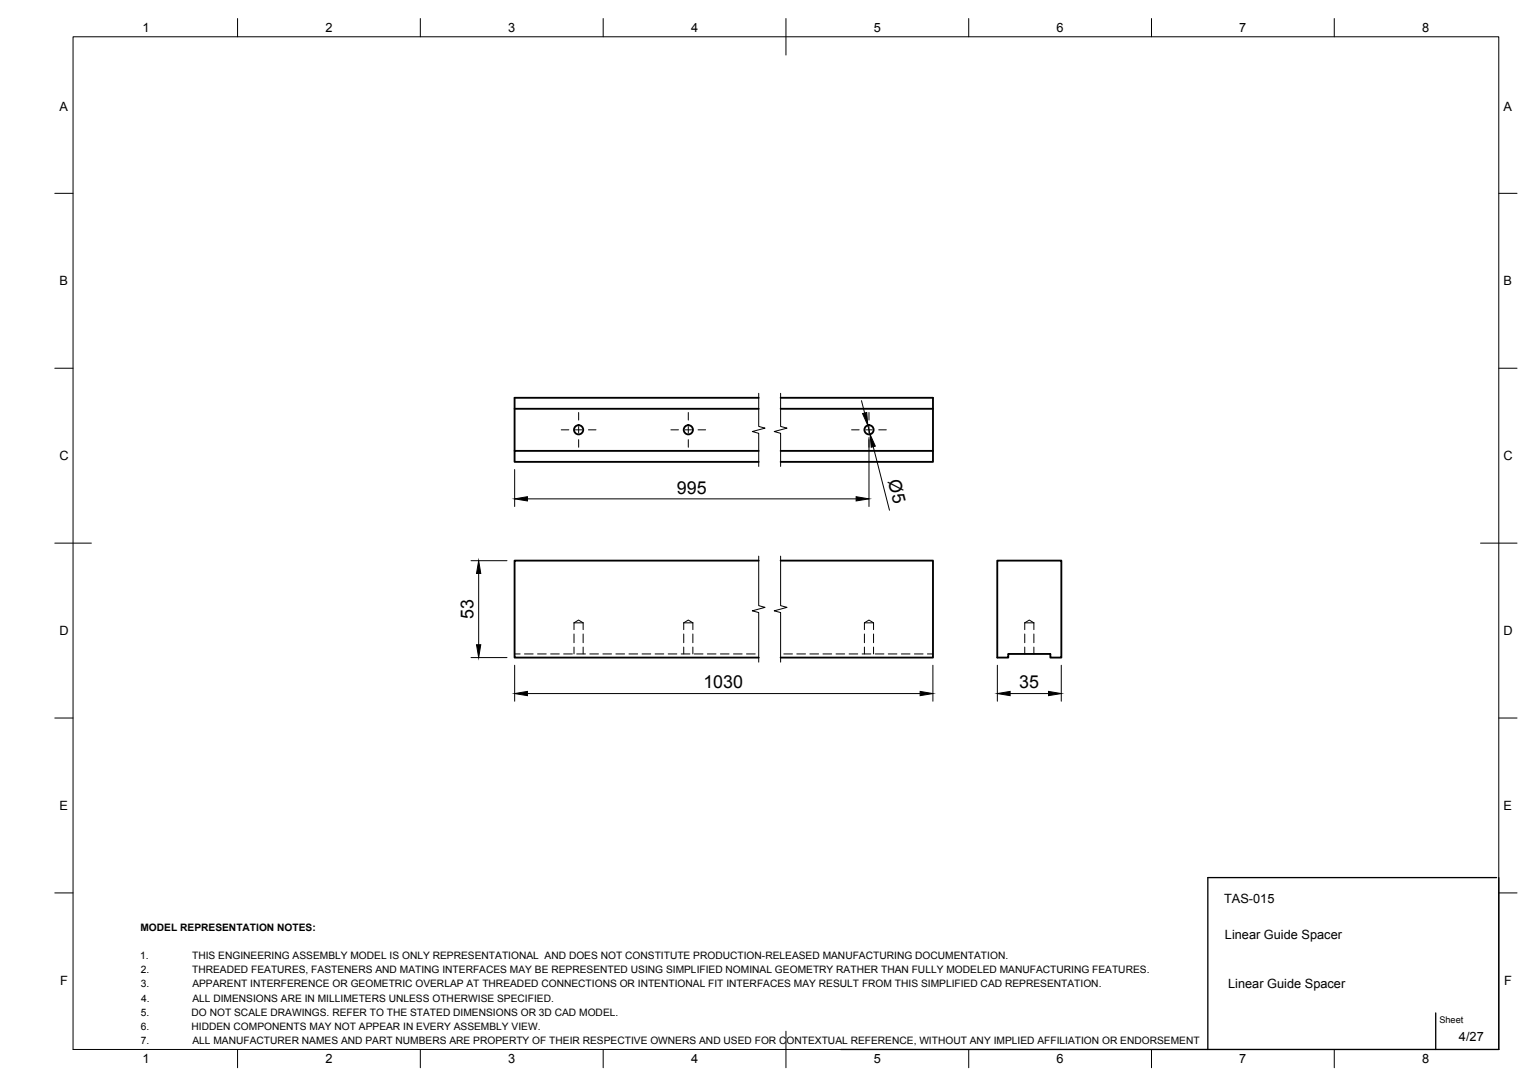
ISO-10303-21;
HEADER;
/* Generated by software containing ST-Developer
 * from STEP Tools, Inc. (www.steptools.com) 
 */

FILE_DESCRIPTION(
/* description */ ('STEP AP214'),
/* implementation_level */ '2;1');

FILE_NAME(
/* name */ 'Linear Guide Spacer.step',
/* time_stamp */ '2026-11-15T14:49:54-08:00',
/* author */ (''),
/* organization */ (''),
/* preprocessor_version */ 'ST-DEVELOPER v20.2',
/* originating_system */ 'Autodesk Translation Framework v15.17.0.0',
/* authorisation */ '');

FILE_SCHEMA (('AUTOMOTIVE_DESIGN { 1 0 10303 214 3 1 1 }'));
ENDSEC;

DATA;
#10=MECHANICAL_DESIGN_GEOMETRIC_PRESENTATION_REPRESENTATION('',(#1126),#66721);
#559=CONICAL_SURFACE('',#28483,2.5,1.02974425867665);
#560=CONICAL_SURFACE('',#28487,2.5,1.02974425867665);
#561=CONICAL_SURFACE('',#28491,2.5,1.02974425867665);
#562=CONICAL_SURFACE('',#28495,2.5,1.02974425867665);
#563=CONICAL_SURFACE('',#28499,2.5,1.02974425867665);
#564=CONICAL_SURFACE('',#28503,2.5,1.02974425867665);
#565=CONICAL_SURFACE('',#28507,2.5,1.02974425867665);
#566=CONICAL_SURFACE('',#28511,2.5,1.02974425867665);
#567=CONICAL_SURFACE('',#28515,2.5,1.02974425867665);
#568=CONICAL_SURFACE('',#28519,2.5,1.02974425867665);
#569=CONICAL_SURFACE('',#28523,2.5,1.02974425867665);
#570=CONICAL_SURFACE('',#28527,2.5,1.02974425867665);
#571=CONICAL_SURFACE('',#28531,2.5,1.02974425867665);
#572=CONICAL_SURFACE('',#28535,2.5,1.02974425867665);
#573=CONICAL_SURFACE('',#28539,2.5,1.02974425867665);
#574=CONICAL_SURFACE('',#28543,2.5,1.02974425867665);
#575=CONICAL_SURFACE('',#28547,2.5,1.02974425867665);
#1062=SHAPE_REPRESENTATION_RELATIONSHIP('SRR','None',#66925,#1093);
#1093=ADVANCED_BREP_SHAPE_REPRESENTATION('',(#1161),#66716);
#1126=STYLED_ITEM('',(#67095),#1161);
#1161=MANIFOLD_SOLID_BREP('Body1',#25692);
#1452=FACE_BOUND('',#5357,.T.);
#1453=FACE_BOUND('',#5358,.T.);
#1454=FACE_BOUND('',#5359,.T.);
#1455=FACE_BOUND('',#5360,.T.);
#1456=FACE_BOUND('',#5361,.T.);
#1457=FACE_BOUND('',#5362,.T.);
#1458=FACE_BOUND('',#5363,.T.);
#1459=FACE_BOUND('',#5364,.T.);
#1460=FACE_BOUND('',#5365,.T.);
#1461=FACE_BOUND('',#5366,.T.);
#1462=FACE_BOUND('',#5367,.T.);
#1463=FACE_BOUND('',#5368,.T.);
#1464=FACE_BOUND('',#5369,.T.);
#1465=FACE_BOUND('',#5370,.T.);
#1466=FACE_BOUND('',#5371,.T.);
#1467=FACE_BOUND('',#5372,.T.);
#1468=FACE_BOUND('',#5373,.T.);
#2209=PLANE('',#28548);
#2210=PLANE('',#28549);
#2211=PLANE('',#28552);
#2212=PLANE('',#28553);
#2213=PLANE('',#28556);
#2214=PLANE('',#28557);
#2215=PLANE('',#28558);
#2216=PLANE('',#28559);
#2217=PLANE('',#28560);
#2218=PLANE('',#28561);
#3588=FACE_OUTER_BOUND('',#5314,.T.);
#3589=FACE_OUTER_BOUND('',#5315,.T.);
#3590=FACE_OUTER_BOUND('',#5316,.T.);
#3591=FACE_OUTER_BOUND('',#5317,.T.);
#3592=FACE_OUTER_BOUND('',#5318,.T.);
#3593=FACE_OUTER_BOUND('',#5319,.T.);
#3594=FACE_OUTER_BOUND('',#5320,.T.);
#3595=FACE_OUTER_BOUND('',#5321,.T.);
#3596=FACE_OUTER_BOUND('',#5322,.T.);
#3597=FACE_OUTER_BOUND('',#5323,.T.);
#3598=FACE_OUTER_BOUND('',#5324,.T.);
#3599=FACE_OUTER_BOUND('',#5325,.T.);
#3600=FACE_OUTER_BOUND('',#5326,.T.);
#3601=FACE_OUTER_BOUND('',#5327,.T.);
#3602=FACE_OUTER_BOUND('',#5328,.T.);
#3603=FACE_OUTER_BOUND('',#5329,.T.);
#3604=FACE_OUTER_BOUND('',#5330,.T.);
#3605=FACE_OUTER_BOUND('',#5331,.T.);
#3606=FACE_OUTER_BOUND('',#5332,.T.);
#3607=FACE_OUTER_BOUND('',#5333,.T.);
#3608=FACE_OUTER_BOUND('',#5334,.T.);
#3609=FACE_OUTER_BOUND('',#5335,.T.);
#3610=FACE_OUTER_BOUND('',#5336,.T.);
#3611=FACE_OUTER_BOUND('',#5337,.T.);
#3612=FACE_OUTER_BOUND('',#5338,.T.);
#3613=FACE_OUTER_BOUND('',#5339,.T.);
#3614=FACE_OUTER_BOUND('',#5340,.T.);
#3615=FACE_OUTER_BOUND('',#5341,.T.);
#3616=FACE_OUTER_BOUND('',#5342,.T.);
#3617=FACE_OUTER_BOUND('',#5343,.T.);
#3618=FACE_OUTER_BOUND('',#5344,.T.);
#3619=FACE_OUTER_BOUND('',#5345,.T.);
#3620=FACE_OUTER_BOUND('',#5346,.T.);
#3621=FACE_OUTER_BOUND('',#5347,.T.);
#3622=FACE_OUTER_BOUND('',#5348,.T.);
#3623=FACE_OUTER_BOUND('',#5349,.T.);
#3624=FACE_OUTER_BOUND('',#5350,.T.);
#3625=FACE_OUTER_BOUND('',#5351,.T.);
#3626=FACE_OUTER_BOUND('',#5352,.T.);
#3627=FACE_OUTER_BOUND('',#5353,.T.);
#3628=FACE_OUTER_BOUND('',#5354,.T.);
#3629=FACE_OUTER_BOUND('',#5355,.T.);
#3630=FACE_OUTER_BOUND('',#5356,.T.);
#3631=FACE_OUTER_BOUND('',#5374,.T.);
#3632=FACE_OUTER_BOUND('',#5375,.T.);
#3633=FACE_OUTER_BOUND('',#5376,.T.);
#5314=EDGE_LOOP('',(#23270,#23271,#23272,#23273));
#5315=EDGE_LOOP('',(#23274,#23275,#23276));
#5316=EDGE_LOOP('',(#23277,#23278,#23279,#23280));
#5317=EDGE_LOOP('',(#23281,#23282,#23283));
#5318=EDGE_LOOP('',(#23284,#23285,#23286,#23287));
#5319=EDGE_LOOP('',(#23288,#23289,#23290));
#5320=EDGE_LOOP('',(#23291,#23292,#23293,#23294));
#5321=EDGE_LOOP('',(#23295,#23296,#23297));
#5322=EDGE_LOOP('',(#23298,#23299,#23300,#23301));
#5323=EDGE_LOOP('',(#23302,#23303,#23304));
#5324=EDGE_LOOP('',(#23305,#23306,#23307,#23308));
#5325=EDGE_LOOP('',(#23309,#23310,#23311));
#5326=EDGE_LOOP('',(#23312,#23313,#23314,#23315));
#5327=EDGE_LOOP('',(#23316,#23317,#23318));
#5328=EDGE_LOOP('',(#23319,#23320,#23321,#23322));
#5329=EDGE_LOOP('',(#23323,#23324,#23325));
#5330=EDGE_LOOP('',(#23326,#23327,#23328,#23329));
#5331=EDGE_LOOP('',(#23330,#23331,#23332));
#5332=EDGE_LOOP('',(#23333,#23334,#23335,#23336));
#5333=EDGE_LOOP('',(#23337,#23338,#23339));
#5334=EDGE_LOOP('',(#23340,#23341,#23342,#23343));
#5335=EDGE_LOOP('',(#23344,#23345,#23346));
#5336=EDGE_LOOP('',(#23347,#23348,#23349,#23350));
#5337=EDGE_LOOP('',(#23351,#23352,#23353));
#5338=EDGE_LOOP('',(#23354,#23355,#23356,#23357));
#5339=EDGE_LOOP('',(#23358,#23359,#23360));
#5340=EDGE_LOOP('',(#23361,#23362,#23363,#23364));
#5341=EDGE_LOOP('',(#23365,#23366,#23367));
#5342=EDGE_LOOP('',(#23368,#23369,#23370,#23371));
#5343=EDGE_LOOP('',(#23372,#23373,#23374));
#5344=EDGE_LOOP('',(#23375,#23376,#23377,#23378));
#5345=EDGE_LOOP('',(#23379,#23380,#23381));
#5346=EDGE_LOOP('',(#23382,#23383,#23384,#23385));
#5347=EDGE_LOOP('',(#23386,#23387,#23388));
#5348=EDGE_LOOP('',(#23389,#23390,#23391,#23392));
#5349=EDGE_LOOP('',(#23393,#23394,#23395,#23396,#23397,#23398,#23399,#23400,
#23401,#23402));
#5350=EDGE_LOOP('',(#23403,#23404,#23405,#23406));
#5351=EDGE_LOOP('',(#23407,#23408,#23409,#23410,#23411,#23412,#23413,#23414,
#23415,#23416));
#5352=EDGE_LOOP('',(#23417,#23418,#23419,#23420));
#5353=EDGE_LOOP('',(#23421,#23422,#23423,#23424));
#5354=EDGE_LOOP('',(#23425,#23426,#23427,#23428));
#5355=EDGE_LOOP('',(#23429,#23430,#23431,#23432));
#5356=EDGE_LOOP('',(#23433,#23434,#23435,#23436));
#5357=EDGE_LOOP('',(#23437));
#5358=EDGE_LOOP('',(#23438));
#5359=EDGE_LOOP('',(#23439));
#5360=EDGE_LOOP('',(#23440));
#5361=EDGE_LOOP('',(#23441));
#5362=EDGE_LOOP('',(#23442));
#5363=EDGE_LOOP('',(#23443));
#5364=EDGE_LOOP('',(#23444));
#5365=EDGE_LOOP('',(#23445));
#5366=EDGE_LOOP('',(#23446));
#5367=EDGE_LOOP('',(#23447));
#5368=EDGE_LOOP('',(#23448));
#5369=EDGE_LOOP('',(#23449));
#5370=EDGE_LOOP('',(#23450));
#5371=EDGE_LOOP('',(#23451));
#5372=EDGE_LOOP('',(#23452));
#5373=EDGE_LOOP('',(#23453));
#5374=EDGE_LOOP('',(#23454,#23455,#23456,#23457));
#5375=EDGE_LOOP('',(#23458,#23459,#23460,#23461));
#5376=EDGE_LOOP('',(#23462,#23463,#23464,#23465));
#7301=LINE('',#66016,#9290);
#7302=LINE('',#66020,#9291);
#7303=LINE('',#66025,#9292);
#7304=LINE('',#66029,#9293);
#7305=LINE('',#66034,#9294);
#7306=LINE('',#66038,#9295);
#7307=LINE('',#66043,#9296);
#7308=LINE('',#66047,#9297);
#7309=LINE('',#66052,#9298);
#7310=LINE('',#66056,#9299);
#7311=LINE('',#66061,#9300);
#7312=LINE('',#66065,#9301);
#7313=LINE('',#66070,#9302);
#7314=LINE('',#66074,#9303);
#7315=LINE('',#66079,#9304);
#7316=LINE('',#66083,#9305);
#7317=LINE('',#66088,#9306);
#7318=LINE('',#66092,#9307);
#7319=LINE('',#66097,#9308);
#7320=LINE('',#66101,#9309);
#7321=LINE('',#66106,#9310);
#7322=LINE('',#66110,#9311);
#7323=LINE('',#66115,#9312);
#7324=LINE('',#66119,#9313);
#7325=LINE('',#66124,#9314);
#7326=LINE('',#66128,#9315);
#7327=LINE('',#66133,#9316);
#7328=LINE('',#66137,#9317);
#7329=LINE('',#66142,#9318);
#7330=LINE('',#66146,#9319);
#7331=LINE('',#66151,#9320);
#7332=LINE('',#66155,#9321);
#7333=LINE('',#66160,#9322);
#7334=LINE('',#66164,#9323);
#7335=LINE('',#66168,#9324);
#7336=LINE('',#66170,#9325);
#7337=LINE('',#66172,#9326);
#7338=LINE('',#66173,#9327);
#7339=LINE('',#66176,#9328);
#7340=LINE('',#66180,#9329);
#7341=LINE('',#66184,#9330);
#7342=LINE('',#66186,#9331);
#7343=LINE('',#66188,#9332);
#7344=LINE('',#66190,#9333);
#7345=LINE('',#66191,#9334);
#7346=LINE('',#66194,#9335);
#7347=LINE('',#66196,#9336);
#7348=LINE('',#66197,#9337);
#7349=LINE('',#66201,#9338);
#7350=LINE('',#66205,#9339);
#7351=LINE('',#66208,#9340);
#7352=LINE('',#66209,#9341);
#7353=LINE('',#66211,#9342);
#7354=LINE('',#66212,#9343);
#7355=LINE('',#66214,#9344);
#7356=LINE('',#66215,#9345);
#7357=LINE('',#66219,#9346);
#7358=LINE('',#66221,#9347);
#7359=LINE('',#66222,#9348);
#7360=LINE('',#66224,#9349);
#9290=VECTOR('',#35456,2.5);
#9291=VECTOR('',#35461,2.5);
#9292=VECTOR('',#35466,2.5);
#9293=VECTOR('',#35471,2.5);
#9294=VECTOR('',#35476,2.5);
#9295=VECTOR('',#35481,2.5);
#9296=VECTOR('',#35486,2.5);
#9297=VECTOR('',#35491,2.5);
#9298=VECTOR('',#35496,2.5);
#9299=VECTOR('',#35501,2.5);
#9300=VECTOR('',#35506,2.5);
#9301=VECTOR('',#35511,2.5);
#9302=VECTOR('',#35516,2.5);
#9303=VECTOR('',#35521,2.5);
#9304=VECTOR('',#35526,2.5);
#9305=VECTOR('',#35531,2.5);
#9306=VECTOR('',#35536,2.5);
#9307=VECTOR('',#35541,2.5);
#9308=VECTOR('',#35546,2.5);
#9309=VECTOR('',#35551,2.5);
#9310=VECTOR('',#35556,2.5);
#9311=VECTOR('',#35561,2.5);
#9312=VECTOR('',#35566,2.5);
#9313=VECTOR('',#35571,2.5);
#9314=VECTOR('',#35576,2.5);
#9315=VECTOR('',#35581,2.5);
#9316=VECTOR('',#35586,2.5);
#9317=VECTOR('',#35591,2.5);
#9318=VECTOR('',#35596,2.5);
#9319=VECTOR('',#35601,2.5);
#9320=VECTOR('',#35606,2.5);
#9321=VECTOR('',#35611,2.5);
#9322=VECTOR('',#35616,2.5);
#9323=VECTOR('',#35621,2.5);
#9324=VECTOR('',#35624,1000.);
#9325=VECTOR('',#35625,1000.);
#9326=VECTOR('',#35626,1000.);
#9327=VECTOR('',#35627,1000.);
#9328=VECTOR('',#35630,1000.);
#9329=VECTOR('',#35633,1000.);
#9330=VECTOR('',#35636,1000.);
#9331=VECTOR('',#35637,1000.);
#9332=VECTOR('',#35638,1000.);
#9333=VECTOR('',#35639,1000.);
#9334=VECTOR('',#35640,1000.);
#9335=VECTOR('',#35643,1000.);
#9336=VECTOR('',#35644,1000.);
#9337=VECTOR('',#35645,1000.);
#9338=VECTOR('',#35648,1000.);
#9339=VECTOR('',#35651,1000.);
#9340=VECTOR('',#35654,1000.);
#9341=VECTOR('',#35655,1000.);
#9342=VECTOR('',#35656,1000.);
#9343=VECTOR('',#35657,1000.);
#9344=VECTOR('',#35660,1000.);
#9345=VECTOR('',#35661,1000.);
#9346=VECTOR('',#35668,1000.);
#9347=VECTOR('',#35671,1000.);
#9348=VECTOR('',#35672,1000.);
#9349=VECTOR('',#35675,1000.);
#10543=CIRCLE('',#28481,2.5);
#10544=CIRCLE('',#28482,2.5);
#10545=CIRCLE('',#28485,2.5);
#10546=CIRCLE('',#28486,2.5);
#10547=CIRCLE('',#28489,2.5);
#10548=CIRCLE('',#28490,2.5);
#10549=CIRCLE('',#28493,2.5);
#10550=CIRCLE('',#28494,2.5);
#10551=CIRCLE('',#28497,2.5);
#10552=CIRCLE('',#28498,2.5);
#10553=CIRCLE('',#28501,2.5);
#10554=CIRCLE('',#28502,2.5);
#10555=CIRCLE('',#28505,2.5);
#10556=CIRCLE('',#28506,2.5);
#10557=CIRCLE('',#28509,2.5);
#10558=CIRCLE('',#28510,2.5);
#10559=CIRCLE('',#28513,2.5);
#10560=CIRCLE('',#28514,2.5);
#10561=CIRCLE('',#28517,2.5);
#10562=CIRCLE('',#28518,2.5);
#10563=CIRCLE('',#28521,2.5);
#10564=CIRCLE('',#28522,2.5);
#10565=CIRCLE('',#28525,2.5);
#10566=CIRCLE('',#28526,2.5);
#10567=CIRCLE('',#28529,2.5);
#10568=CIRCLE('',#28530,2.5);
#10569=CIRCLE('',#28533,2.5);
#10570=CIRCLE('',#28534,2.5);
#10571=CIRCLE('',#28537,2.5);
#10572=CIRCLE('',#28538,2.5);
#10573=CIRCLE('',#28541,2.5);
#10574=CIRCLE('',#28542,2.5);
#10575=CIRCLE('',#28545,2.5);
#10576=CIRCLE('',#28546,2.5);
#10577=CIRCLE('',#28550,0.200000000000001);
#10578=CIRCLE('',#28551,0.200000000000001);
#10579=CIRCLE('',#28554,0.200000000000001);
#10580=CIRCLE('',#28555,0.200000000000001);
#12809=VERTEX_POINT('',#66013);
#12810=VERTEX_POINT('',#66015);
#12811=VERTEX_POINT('',#66019);
#12812=VERTEX_POINT('',#66022);
#12813=VERTEX_POINT('',#66024);
#12814=VERTEX_POINT('',#66028);
#12815=VERTEX_POINT('',#66031);
#12816=VERTEX_POINT('',#66033);
#12817=VERTEX_POINT('',#66037);
#12818=VERTEX_POINT('',#66040);
#12819=VERTEX_POINT('',#66042);
#12820=VERTEX_POINT('',#66046);
#12821=VERTEX_POINT('',#66049);
#12822=VERTEX_POINT('',#66051);
#12823=VERTEX_POINT('',#66055);
#12824=VERTEX_POINT('',#66058);
#12825=VERTEX_POINT('',#66060);
#12826=VERTEX_POINT('',#66064);
#12827=VERTEX_POINT('',#66067);
#12828=VERTEX_POINT('',#66069);
#12829=VERTEX_POINT('',#66073);
#12830=VERTEX_POINT('',#66076);
#12831=VERTEX_POINT('',#66078);
#12832=VERTEX_POINT('',#66082);
#12833=VERTEX_POINT('',#66085);
#12834=VERTEX_POINT('',#66087);
#12835=VERTEX_POINT('',#66091);
#12836=VERTEX_POINT('',#66094);
#12837=VERTEX_POINT('',#66096);
#12838=VERTEX_POINT('',#66100);
#12839=VERTEX_POINT('',#66103);
#12840=VERTEX_POINT('',#66105);
#12841=VERTEX_POINT('',#66109);
#12842=VERTEX_POINT('',#66112);
#12843=VERTEX_POINT('',#66114);
#12844=VERTEX_POINT('',#66118);
#12845=VERTEX_POINT('',#66121);
#12846=VERTEX_POINT('',#66123);
#12847=VERTEX_POINT('',#66127);
#12848=VERTEX_POINT('',#66130);
#12849=VERTEX_POINT('',#66132);
#12850=VERTEX_POINT('',#66136);
#12851=VERTEX_POINT('',#66139);
#12852=VERTEX_POINT('',#66141);
#12853=VERTEX_POINT('',#66145);
#12854=VERTEX_POINT('',#66148);
#12855=VERTEX_POINT('',#66150);
#12856=VERTEX_POINT('',#66154);
#12857=VERTEX_POINT('',#66157);
#12858=VERTEX_POINT('',#66159);
#12859=VERTEX_POINT('',#66163);
#12860=VERTEX_POINT('',#66166);
#12861=VERTEX_POINT('',#66167);
#12862=VERTEX_POINT('',#66169);
#12863=VERTEX_POINT('',#66171);
#12864=VERTEX_POINT('',#66175);
#12865=VERTEX_POINT('',#66177);
#12866=VERTEX_POINT('',#66179);
#12867=VERTEX_POINT('',#66181);
#12868=VERTEX_POINT('',#66183);
#12869=VERTEX_POINT('',#66185);
#12870=VERTEX_POINT('',#66187);
#12871=VERTEX_POINT('',#66189);
#12872=VERTEX_POINT('',#66193);
#12873=VERTEX_POINT('',#66195);
#12874=VERTEX_POINT('',#66199);
#12875=VERTEX_POINT('',#66200);
#12876=VERTEX_POINT('',#66202);
#12877=VERTEX_POINT('',#66204);
#12878=VERTEX_POINT('',#66206);
#12879=VERTEX_POINT('',#66210);
#16328=EDGE_CURVE('',#12809,#12809,#10543,.T.);
#16329=EDGE_CURVE('',#12809,#12810,#7301,.T.);
#16330=EDGE_CURVE('',#12810,#12810,#10544,.T.);
#16331=EDGE_CURVE('',#12811,#12809,#7302,.T.);
#16332=EDGE_CURVE('',#12812,#12812,#10545,.T.);
#16333=EDGE_CURVE('',#12812,#12813,#7303,.T.);
#16334=EDGE_CURVE('',#12813,#12813,#10546,.T.);
#16335=EDGE_CURVE('',#12814,#12812,#7304,.T.);
#16336=EDGE_CURVE('',#12815,#12815,#10547,.T.);
#16337=EDGE_CURVE('',#12815,#12816,#7305,.T.);
#16338=EDGE_CURVE('',#12816,#12816,#10548,.T.);
#16339=EDGE_CURVE('',#12817,#12815,#7306,.T.);
#16340=EDGE_CURVE('',#12818,#12818,#10549,.T.);
#16341=EDGE_CURVE('',#12818,#12819,#7307,.T.);
#16342=EDGE_CURVE('',#12819,#12819,#10550,.T.);
#16343=EDGE_CURVE('',#12820,#12818,#7308,.T.);
#16344=EDGE_CURVE('',#12821,#12821,#10551,.T.);
#16345=EDGE_CURVE('',#12821,#12822,#7309,.T.);
#16346=EDGE_CURVE('',#12822,#12822,#10552,.T.);
#16347=EDGE_CURVE('',#12823,#12821,#7310,.T.);
#16348=EDGE_CURVE('',#12824,#12824,#10553,.T.);
#16349=EDGE_CURVE('',#12824,#12825,#7311,.T.);
#16350=EDGE_CURVE('',#12825,#12825,#10554,.T.);
#16351=EDGE_CURVE('',#12826,#12824,#7312,.T.);
#16352=EDGE_CURVE('',#12827,#12827,#10555,.T.);
#16353=EDGE_CURVE('',#12827,#12828,#7313,.T.);
#16354=EDGE_CURVE('',#12828,#12828,#10556,.T.);
#16355=EDGE_CURVE('',#12829,#12827,#7314,.T.);
#16356=EDGE_CURVE('',#12830,#12830,#10557,.T.);
#16357=EDGE_CURVE('',#12830,#12831,#7315,.T.);
#16358=EDGE_CURVE('',#12831,#12831,#10558,.T.);
#16359=EDGE_CURVE('',#12832,#12830,#7316,.T.);
#16360=EDGE_CURVE('',#12833,#12833,#10559,.T.);
#16361=EDGE_CURVE('',#12833,#12834,#7317,.T.);
#16362=EDGE_CURVE('',#12834,#12834,#10560,.T.);
#16363=EDGE_CURVE('',#12835,#12833,#7318,.T.);
#16364=EDGE_CURVE('',#12836,#12836,#10561,.T.);
#16365=EDGE_CURVE('',#12836,#12837,#7319,.T.);
#16366=EDGE_CURVE('',#12837,#12837,#10562,.T.);
#16367=EDGE_CURVE('',#12838,#12836,#7320,.T.);
#16368=EDGE_CURVE('',#12839,#12839,#10563,.T.);
#16369=EDGE_CURVE('',#12839,#12840,#7321,.T.);
#16370=EDGE_CURVE('',#12840,#12840,#10564,.T.);
#16371=EDGE_CURVE('',#12841,#12839,#7322,.T.);
#16372=EDGE_CURVE('',#12842,#12842,#10565,.T.);
#16373=EDGE_CURVE('',#12842,#12843,#7323,.T.);
#16374=EDGE_CURVE('',#12843,#12843,#10566,.T.);
#16375=EDGE_CURVE('',#12844,#12842,#7324,.T.);
#16376=EDGE_CURVE('',#12845,#12845,#10567,.T.);
#16377=EDGE_CURVE('',#12845,#12846,#7325,.T.);
#16378=EDGE_CURVE('',#12846,#12846,#10568,.T.);
#16379=EDGE_CURVE('',#12847,#12845,#7326,.T.);
#16380=EDGE_CURVE('',#12848,#12848,#10569,.T.);
#16381=EDGE_CURVE('',#12848,#12849,#7327,.T.);
#16382=EDGE_CURVE('',#12849,#12849,#10570,.T.);
#16383=EDGE_CURVE('',#12850,#12848,#7328,.T.);
#16384=EDGE_CURVE('',#12851,#12851,#10571,.T.);
#16385=EDGE_CURVE('',#12851,#12852,#7329,.T.);
#16386=EDGE_CURVE('',#12852,#12852,#10572,.T.);
#16387=EDGE_CURVE('',#12853,#12851,#7330,.T.);
#16388=EDGE_CURVE('',#12854,#12854,#10573,.T.);
#16389=EDGE_CURVE('',#12854,#12855,#7331,.T.);
#16390=EDGE_CURVE('',#12855,#12855,#10574,.T.);
#16391=EDGE_CURVE('',#12856,#12854,#7332,.T.);
#16392=EDGE_CURVE('',#12857,#12857,#10575,.T.);
#16393=EDGE_CURVE('',#12857,#12858,#7333,.T.);
#16394=EDGE_CURVE('',#12858,#12858,#10576,.T.);
#16395=EDGE_CURVE('',#12859,#12857,#7334,.T.);
#16396=EDGE_CURVE('',#12860,#12861,#7335,.T.);
#16397=EDGE_CURVE('',#12861,#12862,#7336,.T.);
#16398=EDGE_CURVE('',#12863,#12862,#7337,.T.);
#16399=EDGE_CURVE('',#12860,#12863,#7338,.T.);
#16400=EDGE_CURVE('',#12864,#12862,#7339,.T.);
#16401=EDGE_CURVE('',#12864,#12865,#10577,.T.);
#16402=EDGE_CURVE('',#12866,#12865,#7340,.T.);
#16403=EDGE_CURVE('',#12866,#12867,#10578,.T.);
#16404=EDGE_CURVE('',#12868,#12867,#7341,.T.);
#16405=EDGE_CURVE('',#12868,#12869,#7342,.T.);
#16406=EDGE_CURVE('',#12869,#12870,#7343,.T.);
#16407=EDGE_CURVE('',#12871,#12870,#7344,.T.);
#16408=EDGE_CURVE('',#12863,#12871,#7345,.T.);
#16409=EDGE_CURVE('',#12870,#12872,#7346,.T.);
#16410=EDGE_CURVE('',#12873,#12872,#7347,.T.);
#16411=EDGE_CURVE('',#12871,#12873,#7348,.T.);
#16412=EDGE_CURVE('',#12874,#12875,#7349,.T.);
#16413=EDGE_CURVE('',#12875,#12876,#10579,.T.);
#16414=EDGE_CURVE('',#12876,#12877,#7350,.T.);
#16415=EDGE_CURVE('',#12877,#12878,#10580,.T.);
#16416=EDGE_CURVE('',#12878,#12861,#7351,.T.);
#16417=EDGE_CURVE('',#12873,#12860,#7352,.T.);
#16418=EDGE_CURVE('',#12872,#12879,#7353,.T.);
#16419=EDGE_CURVE('',#12874,#12879,#7354,.T.);
#16420=EDGE_CURVE('',#12874,#12868,#7355,.T.);
#16421=EDGE_CURVE('',#12879,#12869,#7356,.T.);
#16422=EDGE_CURVE('',#12878,#12864,#7357,.T.);
#16423=EDGE_CURVE('',#12876,#12866,#7358,.T.);
#16424=EDGE_CURVE('',#12865,#12877,#7359,.T.);
#16425=EDGE_CURVE('',#12867,#12875,#7360,.T.);
#23270=ORIENTED_EDGE('',*,*,#16328,.F.);
#23271=ORIENTED_EDGE('',*,*,#16329,.T.);
#23272=ORIENTED_EDGE('',*,*,#16330,.T.);
#23273=ORIENTED_EDGE('',*,*,#16329,.F.);
#23274=ORIENTED_EDGE('',*,*,#16331,.T.);
#23275=ORIENTED_EDGE('',*,*,#16328,.T.);
#23276=ORIENTED_EDGE('',*,*,#16331,.F.);
#23277=ORIENTED_EDGE('',*,*,#16332,.F.);
#23278=ORIENTED_EDGE('',*,*,#16333,.T.);
#23279=ORIENTED_EDGE('',*,*,#16334,.T.);
#23280=ORIENTED_EDGE('',*,*,#16333,.F.);
#23281=ORIENTED_EDGE('',*,*,#16335,.T.);
#23282=ORIENTED_EDGE('',*,*,#16332,.T.);
#23283=ORIENTED_EDGE('',*,*,#16335,.F.);
#23284=ORIENTED_EDGE('',*,*,#16336,.F.);
#23285=ORIENTED_EDGE('',*,*,#16337,.T.);
#23286=ORIENTED_EDGE('',*,*,#16338,.T.);
#23287=ORIENTED_EDGE('',*,*,#16337,.F.);
#23288=ORIENTED_EDGE('',*,*,#16339,.T.);
#23289=ORIENTED_EDGE('',*,*,#16336,.T.);
#23290=ORIENTED_EDGE('',*,*,#16339,.F.);
#23291=ORIENTED_EDGE('',*,*,#16340,.F.);
#23292=ORIENTED_EDGE('',*,*,#16341,.T.);
#23293=ORIENTED_EDGE('',*,*,#16342,.T.);
#23294=ORIENTED_EDGE('',*,*,#16341,.F.);
#23295=ORIENTED_EDGE('',*,*,#16343,.T.);
#23296=ORIENTED_EDGE('',*,*,#16340,.T.);
#23297=ORIENTED_EDGE('',*,*,#16343,.F.);
#23298=ORIENTED_EDGE('',*,*,#16344,.F.);
#23299=ORIENTED_EDGE('',*,*,#16345,.T.);
#23300=ORIENTED_EDGE('',*,*,#16346,.T.);
#23301=ORIENTED_EDGE('',*,*,#16345,.F.);
#23302=ORIENTED_EDGE('',*,*,#16347,.T.);
#23303=ORIENTED_EDGE('',*,*,#16344,.T.);
#23304=ORIENTED_EDGE('',*,*,#16347,.F.);
#23305=ORIENTED_EDGE('',*,*,#16348,.F.);
#23306=ORIENTED_EDGE('',*,*,#16349,.T.);
#23307=ORIENTED_EDGE('',*,*,#16350,.T.);
#23308=ORIENTED_EDGE('',*,*,#16349,.F.);
#23309=ORIENTED_EDGE('',*,*,#16351,.T.);
#23310=ORIENTED_EDGE('',*,*,#16348,.T.);
#23311=ORIENTED_EDGE('',*,*,#16351,.F.);
#23312=ORIENTED_EDGE('',*,*,#16352,.F.);
#23313=ORIENTED_EDGE('',*,*,#16353,.T.);
#23314=ORIENTED_EDGE('',*,*,#16354,.T.);
#23315=ORIENTED_EDGE('',*,*,#16353,.F.);
#23316=ORIENTED_EDGE('',*,*,#16355,.T.);
#23317=ORIENTED_EDGE('',*,*,#16352,.T.);
#23318=ORIENTED_EDGE('',*,*,#16355,.F.);
#23319=ORIENTED_EDGE('',*,*,#16356,.F.);
#23320=ORIENTED_EDGE('',*,*,#16357,.T.);
#23321=ORIENTED_EDGE('',*,*,#16358,.T.);
#23322=ORIENTED_EDGE('',*,*,#16357,.F.);
#23323=ORIENTED_EDGE('',*,*,#16359,.T.);
#23324=ORIENTED_EDGE('',*,*,#16356,.T.);
#23325=ORIENTED_EDGE('',*,*,#16359,.F.);
#23326=ORIENTED_EDGE('',*,*,#16360,.F.);
#23327=ORIENTED_EDGE('',*,*,#16361,.T.);
#23328=ORIENTED_EDGE('',*,*,#16362,.T.);
#23329=ORIENTED_EDGE('',*,*,#16361,.F.);
#23330=ORIENTED_EDGE('',*,*,#16363,.T.);
#23331=ORIENTED_EDGE('',*,*,#16360,.T.);
#23332=ORIENTED_EDGE('',*,*,#16363,.F.);
#23333=ORIENTED_EDGE('',*,*,#16364,.F.);
#23334=ORIENTED_EDGE('',*,*,#16365,.T.);
#23335=ORIENTED_EDGE('',*,*,#16366,.T.);
#23336=ORIENTED_EDGE('',*,*,#16365,.F.);
#23337=ORIENTED_EDGE('',*,*,#16367,.T.);
#23338=ORIENTED_EDGE('',*,*,#16364,.T.);
#23339=ORIENTED_EDGE('',*,*,#16367,.F.);
#23340=ORIENTED_EDGE('',*,*,#16368,.F.);
#23341=ORIENTED_EDGE('',*,*,#16369,.T.);
#23342=ORIENTED_EDGE('',*,*,#16370,.T.);
#23343=ORIENTED_EDGE('',*,*,#16369,.F.);
#23344=ORIENTED_EDGE('',*,*,#16371,.T.);
#23345=ORIENTED_EDGE('',*,*,#16368,.T.);
#23346=ORIENTED_EDGE('',*,*,#16371,.F.);
#23347=ORIENTED_EDGE('',*,*,#16372,.F.);
#23348=ORIENTED_EDGE('',*,*,#16373,.T.);
#23349=ORIENTED_EDGE('',*,*,#16374,.T.);
#23350=ORIENTED_EDGE('',*,*,#16373,.F.);
#23351=ORIENTED_EDGE('',*,*,#16375,.T.);
#23352=ORIENTED_EDGE('',*,*,#16372,.T.);
#23353=ORIENTED_EDGE('',*,*,#16375,.F.);
#23354=ORIENTED_EDGE('',*,*,#16376,.F.);
#23355=ORIENTED_EDGE('',*,*,#16377,.T.);
#23356=ORIENTED_EDGE('',*,*,#16378,.T.);
#23357=ORIENTED_EDGE('',*,*,#16377,.F.);
#23358=ORIENTED_EDGE('',*,*,#16379,.T.);
#23359=ORIENTED_EDGE('',*,*,#16376,.T.);
#23360=ORIENTED_EDGE('',*,*,#16379,.F.);
#23361=ORIENTED_EDGE('',*,*,#16380,.F.);
#23362=ORIENTED_EDGE('',*,*,#16381,.T.);
#23363=ORIENTED_EDGE('',*,*,#16382,.T.);
#23364=ORIENTED_EDGE('',*,*,#16381,.F.);
#23365=ORIENTED_EDGE('',*,*,#16383,.T.);
#23366=ORIENTED_EDGE('',*,*,#16380,.T.);
#23367=ORIENTED_EDGE('',*,*,#16383,.F.);
#23368=ORIENTED_EDGE('',*,*,#16384,.F.);
#23369=ORIENTED_EDGE('',*,*,#16385,.T.);
#23370=ORIENTED_EDGE('',*,*,#16386,.T.);
#23371=ORIENTED_EDGE('',*,*,#16385,.F.);
#23372=ORIENTED_EDGE('',*,*,#16387,.T.);
#23373=ORIENTED_EDGE('',*,*,#16384,.T.);
#23374=ORIENTED_EDGE('',*,*,#16387,.F.);
#23375=ORIENTED_EDGE('',*,*,#16388,.F.);
#23376=ORIENTED_EDGE('',*,*,#16389,.T.);
#23377=ORIENTED_EDGE('',*,*,#16390,.T.);
#23378=ORIENTED_EDGE('',*,*,#16389,.F.);
#23379=ORIENTED_EDGE('',*,*,#16391,.T.);
#23380=ORIENTED_EDGE('',*,*,#16388,.T.);
#23381=ORIENTED_EDGE('',*,*,#16391,.F.);
#23382=ORIENTED_EDGE('',*,*,#16392,.F.);
#23383=ORIENTED_EDGE('',*,*,#16393,.T.);
#23384=ORIENTED_EDGE('',*,*,#16394,.T.);
#23385=ORIENTED_EDGE('',*,*,#16393,.F.);
#23386=ORIENTED_EDGE('',*,*,#16395,.T.);
#23387=ORIENTED_EDGE('',*,*,#16392,.T.);
#23388=ORIENTED_EDGE('',*,*,#16395,.F.);
#23389=ORIENTED_EDGE('',*,*,#16396,.T.);
#23390=ORIENTED_EDGE('',*,*,#16397,.T.);
#23391=ORIENTED_EDGE('',*,*,#16398,.F.);
#23392=ORIENTED_EDGE('',*,*,#16399,.F.);
#23393=ORIENTED_EDGE('',*,*,#16398,.T.);
#23394=ORIENTED_EDGE('',*,*,#16400,.F.);
#23395=ORIENTED_EDGE('',*,*,#16401,.T.);
#23396=ORIENTED_EDGE('',*,*,#16402,.F.);
#23397=ORIENTED_EDGE('',*,*,#16403,.T.);
#23398=ORIENTED_EDGE('',*,*,#16404,.F.);
#23399=ORIENTED_EDGE('',*,*,#16405,.T.);
#23400=ORIENTED_EDGE('',*,*,#16406,.T.);
#23401=ORIENTED_EDGE('',*,*,#16407,.F.);
#23402=ORIENTED_EDGE('',*,*,#16408,.F.);
#23403=ORIENTED_EDGE('',*,*,#16409,.T.);
#23404=ORIENTED_EDGE('',*,*,#16410,.F.);
#23405=ORIENTED_EDGE('',*,*,#16411,.F.);
#23406=ORIENTED_EDGE('',*,*,#16407,.T.);
#23407=ORIENTED_EDGE('',*,*,#16412,.T.);
#23408=ORIENTED_EDGE('',*,*,#16413,.T.);
#23409=ORIENTED_EDGE('',*,*,#16414,.T.);
#23410=ORIENTED_EDGE('',*,*,#16415,.T.);
#23411=ORIENTED_EDGE('',*,*,#16416,.T.);
#23412=ORIENTED_EDGE('',*,*,#16396,.F.);
#23413=ORIENTED_EDGE('',*,*,#16417,.F.);
#23414=ORIENTED_EDGE('',*,*,#16410,.T.);
#23415=ORIENTED_EDGE('',*,*,#16418,.T.);
#23416=ORIENTED_EDGE('',*,*,#16419,.F.);
#23417=ORIENTED_EDGE('',*,*,#16405,.F.);
#23418=ORIENTED_EDGE('',*,*,#16420,.F.);
#23419=ORIENTED_EDGE('',*,*,#16419,.T.);
#23420=ORIENTED_EDGE('',*,*,#16421,.T.);
#23421=ORIENTED_EDGE('',*,*,#16408,.T.);
#23422=ORIENTED_EDGE('',*,*,#16411,.T.);
#23423=ORIENTED_EDGE('',*,*,#16417,.T.);
#23424=ORIENTED_EDGE('',*,*,#16399,.T.);
#23425=ORIENTED_EDGE('',*,*,#16406,.F.);
#23426=ORIENTED_EDGE('',*,*,#16421,.F.);
#23427=ORIENTED_EDGE('',*,*,#16418,.F.);
#23428=ORIENTED_EDGE('',*,*,#16409,.F.);
#23429=ORIENTED_EDGE('',*,*,#16416,.F.);
#23430=ORIENTED_EDGE('',*,*,#16422,.T.);
#23431=ORIENTED_EDGE('',*,*,#16400,.T.);
#23432=ORIENTED_EDGE('',*,*,#16397,.F.);
#23433=ORIENTED_EDGE('',*,*,#16414,.F.);
#23434=ORIENTED_EDGE('',*,*,#16423,.T.);
#23435=ORIENTED_EDGE('',*,*,#16402,.T.);
#23436=ORIENTED_EDGE('',*,*,#16424,.T.);
#23437=ORIENTED_EDGE('',*,*,#16330,.F.);
#23438=ORIENTED_EDGE('',*,*,#16334,.F.);
#23439=ORIENTED_EDGE('',*,*,#16338,.F.);
#23440=ORIENTED_EDGE('',*,*,#16342,.F.);
#23441=ORIENTED_EDGE('',*,*,#16346,.F.);
#23442=ORIENTED_EDGE('',*,*,#16350,.F.);
#23443=ORIENTED_EDGE('',*,*,#16354,.F.);
#23444=ORIENTED_EDGE('',*,*,#16358,.F.);
#23445=ORIENTED_EDGE('',*,*,#16362,.F.);
#23446=ORIENTED_EDGE('',*,*,#16366,.F.);
#23447=ORIENTED_EDGE('',*,*,#16370,.F.);
#23448=ORIENTED_EDGE('',*,*,#16374,.F.);
#23449=ORIENTED_EDGE('',*,*,#16378,.F.);
#23450=ORIENTED_EDGE('',*,*,#16382,.F.);
#23451=ORIENTED_EDGE('',*,*,#16386,.F.);
#23452=ORIENTED_EDGE('',*,*,#16390,.F.);
#23453=ORIENTED_EDGE('',*,*,#16394,.F.);
#23454=ORIENTED_EDGE('',*,*,#16404,.T.);
#23455=ORIENTED_EDGE('',*,*,#16425,.T.);
#23456=ORIENTED_EDGE('',*,*,#16412,.F.);
#23457=ORIENTED_EDGE('',*,*,#16420,.T.);
#23458=ORIENTED_EDGE('',*,*,#16413,.F.);
#23459=ORIENTED_EDGE('',*,*,#16425,.F.);
#23460=ORIENTED_EDGE('',*,*,#16403,.F.);
#23461=ORIENTED_EDGE('',*,*,#16423,.F.);
#23462=ORIENTED_EDGE('',*,*,#16415,.F.);
#23463=ORIENTED_EDGE('',*,*,#16424,.F.);
#23464=ORIENTED_EDGE('',*,*,#16401,.F.);
#23465=ORIENTED_EDGE('',*,*,#16422,.F.);
#24182=CYLINDRICAL_SURFACE('',#28480,2.5);
#24183=CYLINDRICAL_SURFACE('',#28484,2.5);
#24184=CYLINDRICAL_SURFACE('',#28488,2.5);
#24185=CYLINDRICAL_SURFACE('',#28492,2.5);
#24186=CYLINDRICAL_SURFACE('',#28496,2.5);
#24187=CYLINDRICAL_SURFACE('',#28500,2.5);
#24188=CYLINDRICAL_SURFACE('',#28504,2.5);
#24189=CYLINDRICAL_SURFACE('',#28508,2.5);
#24190=CYLINDRICAL_SURFACE('',#28512,2.5);
#24191=CYLINDRICAL_SURFACE('',#28516,2.5);
#24192=CYLINDRICAL_SURFACE('',#28520,2.5);
#24193=CYLINDRICAL_SURFACE('',#28524,2.5);
#24194=CYLINDRICAL_SURFACE('',#28528,2.5);
#24195=CYLINDRICAL_SURFACE('',#28532,2.5);
#24196=CYLINDRICAL_SURFACE('',#28536,2.5);
#24197=CYLINDRICAL_SURFACE('',#28540,2.5);
#24198=CYLINDRICAL_SURFACE('',#28544,2.5);
#24199=CYLINDRICAL_SURFACE('',#28562,0.200000000000001);
#24200=CYLINDRICAL_SURFACE('',#28563,0.200000000000001);
#25541=ADVANCED_FACE('',(#3588),#24182,.F.);
#25542=ADVANCED_FACE('',(#3589),#559,.F.);
#25543=ADVANCED_FACE('',(#3590),#24183,.F.);
#25544=ADVANCED_FACE('',(#3591),#560,.F.);
#25545=ADVANCED_FACE('',(#3592),#24184,.F.);
#25546=ADVANCED_FACE('',(#3593),#561,.F.);
#25547=ADVANCED_FACE('',(#3594),#24185,.F.);
#25548=ADVANCED_FACE('',(#3595),#562,.F.);
#25549=ADVANCED_FACE('',(#3596),#24186,.F.);
#25550=ADVANCED_FACE('',(#3597),#563,.F.);
#25551=ADVANCED_FACE('',(#3598),#24187,.F.);
#25552=ADVANCED_FACE('',(#3599),#564,.F.);
#25553=ADVANCED_FACE('',(#3600),#24188,.F.);
#25554=ADVANCED_FACE('',(#3601),#565,.F.);
#25555=ADVANCED_FACE('',(#3602),#24189,.F.);
#25556=ADVANCED_FACE('',(#3603),#566,.F.);
#25557=ADVANCED_FACE('',(#3604),#24190,.F.);
#25558=ADVANCED_FACE('',(#3605),#567,.F.);
#25559=ADVANCED_FACE('',(#3606),#24191,.F.);
#25560=ADVANCED_FACE('',(#3607),#568,.F.);
#25561=ADVANCED_FACE('',(#3608),#24192,.F.);
#25562=ADVANCED_FACE('',(#3609),#569,.F.);
#25563=ADVANCED_FACE('',(#3610),#24193,.F.);
#25564=ADVANCED_FACE('',(#3611),#570,.F.);
#25565=ADVANCED_FACE('',(#3612),#24194,.F.);
#25566=ADVANCED_FACE('',(#3613),#571,.F.);
#25567=ADVANCED_FACE('',(#3614),#24195,.F.);
#25568=ADVANCED_FACE('',(#3615),#572,.F.);
#25569=ADVANCED_FACE('',(#3616),#24196,.F.);
#25570=ADVANCED_FACE('',(#3617),#573,.F.);
#25571=ADVANCED_FACE('',(#3618),#24197,.F.);
#25572=ADVANCED_FACE('',(#3619),#574,.F.);
#25573=ADVANCED_FACE('',(#3620),#24198,.F.);
#25574=ADVANCED_FACE('',(#3621),#575,.F.);
#25575=ADVANCED_FACE('',(#3622),#2209,.F.);
#25576=ADVANCED_FACE('',(#3623),#2210,.F.);
#25577=ADVANCED_FACE('',(#3624),#2211,.F.);
#25578=ADVANCED_FACE('',(#3625),#2212,.F.);
#25579=ADVANCED_FACE('',(#3626),#2213,.F.);
#25580=ADVANCED_FACE('',(#3627),#2214,.T.);
#25581=ADVANCED_FACE('',(#3628),#2215,.F.);
#25582=ADVANCED_FACE('',(#3629),#2216,.F.);
#25583=ADVANCED_FACE('',(#3630,#1452,#1453,#1454,#1455,#1456,#1457,#1458,
#1459,#1460,#1461,#1462,#1463,#1464,#1465,#1466,#1467,#1468),#2217,.F.);
#25584=ADVANCED_FACE('',(#3631),#2218,.F.);
#25585=ADVANCED_FACE('',(#3632),#24199,.F.);
#25586=ADVANCED_FACE('',(#3633),#24200,.F.);
#25692=CLOSED_SHELL('',(#25541,#25542,#25543,#25544,#25545,#25546,#25547,
#25548,#25549,#25550,#25551,#25552,#25553,#25554,#25555,#25556,#25557,#25558,
#25559,#25560,#25561,#25562,#25563,#25564,#25565,#25566,#25567,#25568,#25569,
#25570,#25571,#25572,#25573,#25574,#25575,#25576,#25577,#25578,#25579,#25580,
#25581,#25582,#25583,#25584,#25585,#25586));
#28479=AXIS2_PLACEMENT_3D('',#66011,#35450,#35451);
#28480=AXIS2_PLACEMENT_3D('',#66012,#35452,#35453);
#28481=AXIS2_PLACEMENT_3D('',#66014,#35454,#35455);
#28482=AXIS2_PLACEMENT_3D('',#66017,#35457,#35458);
#28483=AXIS2_PLACEMENT_3D('',#66018,#35459,#35460);
#28484=AXIS2_PLACEMENT_3D('',#66021,#35462,#35463);
#28485=AXIS2_PLACEMENT_3D('',#66023,#35464,#35465);
#28486=AXIS2_PLACEMENT_3D('',#66026,#35467,#35468);
#28487=AXIS2_PLACEMENT_3D('',#66027,#35469,#35470);
#28488=AXIS2_PLACEMENT_3D('',#66030,#35472,#35473);
#28489=AXIS2_PLACEMENT_3D('',#66032,#35474,#35475);
#28490=AXIS2_PLACEMENT_3D('',#66035,#35477,#35478);
#28491=AXIS2_PLACEMENT_3D('',#66036,#35479,#35480);
#28492=AXIS2_PLACEMENT_3D('',#66039,#35482,#35483);
#28493=AXIS2_PLACEMENT_3D('',#66041,#35484,#35485);
#28494=AXIS2_PLACEMENT_3D('',#66044,#35487,#35488);
#28495=AXIS2_PLACEMENT_3D('',#66045,#35489,#35490);
#28496=AXIS2_PLACEMENT_3D('',#66048,#35492,#35493);
#28497=AXIS2_PLACEMENT_3D('',#66050,#35494,#35495);
#28498=AXIS2_PLACEMENT_3D('',#66053,#35497,#35498);
#28499=AXIS2_PLACEMENT_3D('',#66054,#35499,#35500);
#28500=AXIS2_PLACEMENT_3D('',#66057,#35502,#35503);
#28501=AXIS2_PLACEMENT_3D('',#66059,#35504,#35505);
#28502=AXIS2_PLACEMENT_3D('',#66062,#35507,#35508);
#28503=AXIS2_PLACEMENT_3D('',#66063,#35509,#35510);
#28504=AXIS2_PLACEMENT_3D('',#66066,#35512,#35513);
#28505=AXIS2_PLACEMENT_3D('',#66068,#35514,#35515);
#28506=AXIS2_PLACEMENT_3D('',#66071,#35517,#35518);
#28507=AXIS2_PLACEMENT_3D('',#66072,#35519,#35520);
#28508=AXIS2_PLACEMENT_3D('',#66075,#35522,#35523);
#28509=AXIS2_PLACEMENT_3D('',#66077,#35524,#35525);
#28510=AXIS2_PLACEMENT_3D('',#66080,#35527,#35528);
#28511=AXIS2_PLACEMENT_3D('',#66081,#35529,#35530);
#28512=AXIS2_PLACEMENT_3D('',#66084,#35532,#35533);
#28513=AXIS2_PLACEMENT_3D('',#66086,#35534,#35535);
#28514=AXIS2_PLACEMENT_3D('',#66089,#35537,#35538);
#28515=AXIS2_PLACEMENT_3D('',#66090,#35539,#35540);
#28516=AXIS2_PLACEMENT_3D('',#66093,#35542,#35543);
#28517=AXIS2_PLACEMENT_3D('',#66095,#35544,#35545);
#28518=AXIS2_PLACEMENT_3D('',#66098,#35547,#35548);
#28519=AXIS2_PLACEMENT_3D('',#66099,#35549,#35550);
#28520=AXIS2_PLACEMENT_3D('',#66102,#35552,#35553);
#28521=AXIS2_PLACEMENT_3D('',#66104,#35554,#35555);
#28522=AXIS2_PLACEMENT_3D('',#66107,#35557,#35558);
#28523=AXIS2_PLACEMENT_3D('',#66108,#35559,#35560);
#28524=AXIS2_PLACEMENT_3D('',#66111,#35562,#35563);
#28525=AXIS2_PLACEMENT_3D('',#66113,#35564,#35565);
#28526=AXIS2_PLACEMENT_3D('',#66116,#35567,#35568);
#28527=AXIS2_PLACEMENT_3D('',#66117,#35569,#35570);
#28528=AXIS2_PLACEMENT_3D('',#66120,#35572,#35573);
#28529=AXIS2_PLACEMENT_3D('',#66122,#35574,#35575);
#28530=AXIS2_PLACEMENT_3D('',#66125,#35577,#35578);
#28531=AXIS2_PLACEMENT_3D('',#66126,#35579,#35580);
#28532=AXIS2_PLACEMENT_3D('',#66129,#35582,#35583);
#28533=AXIS2_PLACEMENT_3D('',#66131,#35584,#35585);
#28534=AXIS2_PLACEMENT_3D('',#66134,#35587,#35588);
#28535=AXIS2_PLACEMENT_3D('',#66135,#35589,#35590);
#28536=AXIS2_PLACEMENT_3D('',#66138,#35592,#35593);
#28537=AXIS2_PLACEMENT_3D('',#66140,#35594,#35595);
#28538=AXIS2_PLACEMENT_3D('',#66143,#35597,#35598);
#28539=AXIS2_PLACEMENT_3D('',#66144,#35599,#35600);
#28540=AXIS2_PLACEMENT_3D('',#66147,#35602,#35603);
#28541=AXIS2_PLACEMENT_3D('',#66149,#35604,#35605);
#28542=AXIS2_PLACEMENT_3D('',#66152,#35607,#35608);
#28543=AXIS2_PLACEMENT_3D('',#66153,#35609,#35610);
#28544=AXIS2_PLACEMENT_3D('',#66156,#35612,#35613);
#28545=AXIS2_PLACEMENT_3D('',#66158,#35614,#35615);
#28546=AXIS2_PLACEMENT_3D('',#66161,#35617,#35618);
#28547=AXIS2_PLACEMENT_3D('',#66162,#35619,#35620);
#28548=AXIS2_PLACEMENT_3D('',#66165,#35622,#35623);
#28549=AXIS2_PLACEMENT_3D('',#66174,#35628,#35629);
#28550=AXIS2_PLACEMENT_3D('',#66178,#35631,#35632);
#28551=AXIS2_PLACEMENT_3D('',#66182,#35634,#35635);
#28552=AXIS2_PLACEMENT_3D('',#66192,#35641,#35642);
#28553=AXIS2_PLACEMENT_3D('',#66198,#35646,#35647);
#28554=AXIS2_PLACEMENT_3D('',#66203,#35649,#35650);
#28555=AXIS2_PLACEMENT_3D('',#66207,#35652,#35653);
#28556=AXIS2_PLACEMENT_3D('',#66213,#35658,#35659);
#28557=AXIS2_PLACEMENT_3D('',#66216,#35662,#35663);
#28558=AXIS2_PLACEMENT_3D('',#66217,#35664,#35665);
#28559=AXIS2_PLACEMENT_3D('',#66218,#35666,#35667);
#28560=AXIS2_PLACEMENT_3D('',#66220,#35669,#35670);
#28561=AXIS2_PLACEMENT_3D('',#66223,#35673,#35674);
#28562=AXIS2_PLACEMENT_3D('',#66225,#35676,#35677);
#28563=AXIS2_PLACEMENT_3D('',#66226,#35678,#35679);
#35450=DIRECTION('axis',(0.,0.,1.));
#35451=DIRECTION('refdir',(1.,0.,0.));
#35452=DIRECTION('center_axis',(0.,-1.,0.));
#35453=DIRECTION('ref_axis',(0.,0.,-1.));
#35454=DIRECTION('center_axis',(0.,-1.,0.));
#35455=DIRECTION('ref_axis',(0.,0.,-1.));
#35456=DIRECTION('',(0.,-1.,0.));
#35457=DIRECTION('center_axis',(0.,-1.,0.));
#35458=DIRECTION('ref_axis',(0.,0.,-1.));
#35459=DIRECTION('center_axis',(0.,-1.,0.));
#35460=DIRECTION('ref_axis',(0.,0.,-1.));
#35461=DIRECTION('',(-1.04972719113862E-16,-0.515038074910054,0.857167300702112));
#35462=DIRECTION('center_axis',(0.,-1.,0.));
#35463=DIRECTION('ref_axis',(0.,0.,-1.));
#35464=DIRECTION('center_axis',(0.,-1.,0.));
#35465=DIRECTION('ref_axis',(0.,0.,-1.));
#35466=DIRECTION('',(0.,-1.,0.));
#35467=DIRECTION('center_axis',(0.,-1.,0.));
#35468=DIRECTION('ref_axis',(0.,0.,-1.));
#35469=DIRECTION('center_axis',(0.,-1.,0.));
#35470=DIRECTION('ref_axis',(0.,0.,-1.));
#35471=DIRECTION('',(-1.04972719113862E-16,-0.515038074910054,0.857167300702112));
#35472=DIRECTION('center_axis',(0.,-1.,0.));
#35473=DIRECTION('ref_axis',(0.,0.,-1.));
#35474=DIRECTION('center_axis',(0.,-1.,0.));
#35475=DIRECTION('ref_axis',(0.,0.,-1.));
#35476=DIRECTION('',(0.,-1.,0.));
#35477=DIRECTION('center_axis',(0.,-1.,0.));
#35478=DIRECTION('ref_axis',(0.,0.,-1.));
#35479=DIRECTION('center_axis',(0.,-1.,0.));
#35480=DIRECTION('ref_axis',(0.,0.,-1.));
#35481=DIRECTION('',(-1.04972719113862E-16,-0.515038074910054,0.857167300702112));
#35482=DIRECTION('center_axis',(0.,-1.,0.));
#35483=DIRECTION('ref_axis',(0.,0.,-1.));
#35484=DIRECTION('center_axis',(0.,-1.,0.));
#35485=DIRECTION('ref_axis',(0.,0.,-1.));
#35486=DIRECTION('',(0.,-1.,0.));
#35487=DIRECTION('center_axis',(0.,-1.,0.));
#35488=DIRECTION('ref_axis',(0.,0.,-1.));
#35489=DIRECTION('center_axis',(0.,-1.,0.));
#35490=DIRECTION('ref_axis',(0.,0.,-1.));
#35491=DIRECTION('',(-1.04972719113862E-16,-0.515038074910054,0.857167300702112));
#35492=DIRECTION('center_axis',(0.,-1.,0.));
#35493=DIRECTION('ref_axis',(0.,0.,-1.));
#35494=DIRECTION('center_axis',(0.,-1.,0.));
#35495=DIRECTION('ref_axis',(0.,0.,-1.));
#35496=DIRECTION('',(0.,-1.,0.));
#35497=DIRECTION('center_axis',(0.,-1.,0.));
#35498=DIRECTION('ref_axis',(0.,0.,-1.));
#35499=DIRECTION('center_axis',(0.,-1.,0.));
#35500=DIRECTION('ref_axis',(0.,0.,-1.));
#35501=DIRECTION('',(-1.04972719113862E-16,-0.515038074910054,0.857167300702112));
#35502=DIRECTION('center_axis',(0.,-1.,0.));
#35503=DIRECTION('ref_axis',(0.,0.,-1.));
#35504=DIRECTION('center_axis',(0.,-1.,0.));
#35505=DIRECTION('ref_axis',(0.,0.,-1.));
#35506=DIRECTION('',(0.,-1.,0.));
#35507=DIRECTION('center_axis',(0.,-1.,0.));
#35508=DIRECTION('ref_axis',(0.,0.,-1.));
#35509=DIRECTION('center_axis',(0.,-1.,0.));
#35510=DIRECTION('ref_axis',(0.,0.,-1.));
#35511=DIRECTION('',(-1.04972719113862E-16,-0.515038074910054,0.857167300702112));
#35512=DIRECTION('center_axis',(0.,-1.,0.));
#35513=DIRECTION('ref_axis',(0.,0.,-1.));
#35514=DIRECTION('center_axis',(0.,-1.,0.));
#35515=DIRECTION('ref_axis',(0.,0.,-1.));
#35516=DIRECTION('',(0.,-1.,0.));
#35517=DIRECTION('center_axis',(0.,-1.,0.));
#35518=DIRECTION('ref_axis',(0.,0.,-1.));
#35519=DIRECTION('center_axis',(0.,-1.,0.));
#35520=DIRECTION('ref_axis',(0.,0.,-1.));
#35521=DIRECTION('',(-1.04972719113862E-16,-0.515038074910054,0.857167300702112));
#35522=DIRECTION('center_axis',(0.,-1.,0.));
#35523=DIRECTION('ref_axis',(0.,0.,-1.));
#35524=DIRECTION('center_axis',(0.,-1.,0.));
#35525=DIRECTION('ref_axis',(0.,0.,-1.));
#35526=DIRECTION('',(0.,-1.,0.));
#35527=DIRECTION('center_axis',(0.,-1.,0.));
#35528=DIRECTION('ref_axis',(0.,0.,-1.));
#35529=DIRECTION('center_axis',(0.,-1.,0.));
#35530=DIRECTION('ref_axis',(0.,0.,-1.));
#35531=DIRECTION('',(-1.04972719113862E-16,-0.515038074910057,0.857167300702111));
#35532=DIRECTION('center_axis',(0.,-1.,0.));
#35533=DIRECTION('ref_axis',(0.,0.,-1.));
#35534=DIRECTION('center_axis',(0.,-1.,0.));
#35535=DIRECTION('ref_axis',(0.,0.,-1.));
#35536=DIRECTION('',(0.,-1.,0.));
#35537=DIRECTION('center_axis',(0.,-1.,0.));
#35538=DIRECTION('ref_axis',(0.,0.,-1.));
#35539=DIRECTION('center_axis',(0.,-1.,0.));
#35540=DIRECTION('ref_axis',(0.,0.,-1.));
#35541=DIRECTION('',(-1.04972719113862E-16,-0.515038074910054,0.857167300702112));
#35542=DIRECTION('center_axis',(0.,-1.,0.));
#35543=DIRECTION('ref_axis',(0.,0.,-1.));
#35544=DIRECTION('center_axis',(0.,-1.,0.));
#35545=DIRECTION('ref_axis',(0.,0.,-1.));
#35546=DIRECTION('',(0.,-1.,0.));
#35547=DIRECTION('center_axis',(0.,-1.,0.));
#35548=DIRECTION('ref_axis',(0.,0.,-1.));
#35549=DIRECTION('center_axis',(0.,-1.,0.));
#35550=DIRECTION('ref_axis',(0.,0.,-1.));
#35551=DIRECTION('',(-1.04972719113862E-16,-0.515038074910054,0.857167300702112));
#35552=DIRECTION('center_axis',(0.,-1.,0.));
#35553=DIRECTION('ref_axis',(0.,0.,-1.));
#35554=DIRECTION('center_axis',(0.,-1.,0.));
#35555=DIRECTION('ref_axis',(0.,0.,-1.));
#35556=DIRECTION('',(0.,-1.,0.));
#35557=DIRECTION('center_axis',(0.,-1.,0.));
#35558=DIRECTION('ref_axis',(0.,0.,-1.));
#35559=DIRECTION('center_axis',(0.,-1.,0.));
#35560=DIRECTION('ref_axis',(0.,0.,-1.));
#35561=DIRECTION('',(-1.04972719113862E-16,-0.515038074910054,0.857167300702112));
#35562=DIRECTION('center_axis',(0.,-1.,0.));
#35563=DIRECTION('ref_axis',(0.,0.,-1.));
#35564=DIRECTION('center_axis',(0.,-1.,0.));
#35565=DIRECTION('ref_axis',(0.,0.,-1.));
#35566=DIRECTION('',(0.,-1.,0.));
#35567=DIRECTION('center_axis',(0.,-1.,0.));
#35568=DIRECTION('ref_axis',(0.,0.,-1.));
#35569=DIRECTION('center_axis',(0.,-1.,0.));
#35570=DIRECTION('ref_axis',(0.,0.,-1.));
#35571=DIRECTION('',(-1.04972719113862E-16,-0.515038074910054,0.857167300702112));
#35572=DIRECTION('center_axis',(0.,-1.,0.));
#35573=DIRECTION('ref_axis',(0.,0.,-1.));
#35574=DIRECTION('center_axis',(0.,-1.,0.));
#35575=DIRECTION('ref_axis',(0.,0.,-1.));
#35576=DIRECTION('',(0.,-1.,0.));
#35577=DIRECTION('center_axis',(0.,-1.,0.));
#35578=DIRECTION('ref_axis',(0.,0.,-1.));
#35579=DIRECTION('center_axis',(0.,-1.,0.));
#35580=DIRECTION('ref_axis',(0.,0.,-1.));
#35581=DIRECTION('',(-1.04972719113862E-16,-0.515038074910054,0.857167300702112));
#35582=DIRECTION('center_axis',(0.,-1.,0.));
#35583=DIRECTION('ref_axis',(0.,0.,-1.));
#35584=DIRECTION('center_axis',(0.,-1.,0.));
#35585=DIRECTION('ref_axis',(0.,0.,-1.));
#35586=DIRECTION('',(0.,-1.,0.));
#35587=DIRECTION('center_axis',(0.,-1.,0.));
#35588=DIRECTION('ref_axis',(0.,0.,-1.));
#35589=DIRECTION('center_axis',(0.,-1.,0.));
#35590=DIRECTION('ref_axis',(0.,0.,-1.));
#35591=DIRECTION('',(-1.04972719113862E-16,-0.515038074910054,0.857167300702112));
#35592=DIRECTION('center_axis',(0.,-1.,0.));
#35593=DIRECTION('ref_axis',(0.,0.,-1.));
#35594=DIRECTION('center_axis',(0.,-1.,0.));
#35595=DIRECTION('ref_axis',(0.,0.,-1.));
#35596=DIRECTION('',(0.,-1.,0.));
#35597=DIRECTION('center_axis',(0.,-1.,0.));
#35598=DIRECTION('ref_axis',(0.,0.,-1.));
#35599=DIRECTION('center_axis',(0.,-1.,0.));
#35600=DIRECTION('ref_axis',(0.,0.,-1.));
#35601=DIRECTION('',(-1.04972719113862E-16,-0.515038074910054,0.857167300702112));
#35602=DIRECTION('center_axis',(0.,-1.,0.));
#35603=DIRECTION('ref_axis',(0.,0.,-1.));
#35604=DIRECTION('center_axis',(0.,-1.,0.));
#35605=DIRECTION('ref_axis',(0.,0.,-1.));
#35606=DIRECTION('',(0.,-1.,0.));
#35607=DIRECTION('center_axis',(0.,-1.,0.));
#35608=DIRECTION('ref_axis',(0.,0.,-1.));
#35609=DIRECTION('center_axis',(0.,-1.,0.));
#35610=DIRECTION('ref_axis',(0.,0.,-1.));
#35611=DIRECTION('',(-1.04972719113862E-16,-0.515038074910057,0.857167300702111));
#35612=DIRECTION('center_axis',(0.,-1.,0.));
#35613=DIRECTION('ref_axis',(0.,0.,-1.));
#35614=DIRECTION('center_axis',(0.,-1.,0.));
#35615=DIRECTION('ref_axis',(0.,0.,-1.));
#35616=DIRECTION('',(0.,-1.,0.));
#35617=DIRECTION('center_axis',(0.,-1.,0.));
#35618=DIRECTION('ref_axis',(0.,0.,-1.));
#35619=DIRECTION('center_axis',(0.,-1.,0.));
#35620=DIRECTION('ref_axis',(0.,0.,-1.));
#35621=DIRECTION('',(-1.04972719113862E-16,-0.515038074910056,0.857167300702111));
#35622=DIRECTION('center_axis',(0.,1.,0.));
#35623=DIRECTION('ref_axis',(0.,0.,1.));
#35624=DIRECTION('',(0.,0.,-1.));
#35625=DIRECTION('',(1.,0.,0.));
#35626=DIRECTION('',(0.,0.,-1.));
#35627=DIRECTION('',(1.,0.,0.));
#35628=DIRECTION('center_axis',(-1.,0.,0.));
#35629=DIRECTION('ref_axis',(0.,0.,1.));
#35630=DIRECTION('',(0.,-1.,0.));
#35631=DIRECTION('center_axis',(-1.,0.,0.));
#35632=DIRECTION('ref_axis',(0.,0.,1.));
#35633=DIRECTION('',(0.,0.,1.));
#35634=DIRECTION('center_axis',(-1.,0.,0.));
#35635=DIRECTION('ref_axis',(0.,0.,1.));
#35636=DIRECTION('',(0.,1.,0.));
#35637=DIRECTION('',(0.,0.,-1.));
#35638=DIRECTION('',(0.,1.,0.));
#35639=DIRECTION('',(0.,0.,-1.));
#35640=DIRECTION('',(0.,1.,0.));
#35641=DIRECTION('center_axis',(0.,-1.,0.));
#35642=DIRECTION('ref_axis',(0.,0.,-1.));
#35643=DIRECTION('',(-1.,0.,0.));
#35644=DIRECTION('',(0.,0.,-1.));
#35645=DIRECTION('',(-1.,0.,0.));
#35646=DIRECTION('center_axis',(1.,0.,0.));
#35647=DIRECTION('ref_axis',(0.,0.,-1.));
#35648=DIRECTION('',(0.,1.,0.));
#35649=DIRECTION('center_axis',(1.,0.,0.));
#35650=DIRECTION('ref_axis',(0.,0.,-1.));
#35651=DIRECTION('',(0.,0.,1.));
#35652=DIRECTION('center_axis',(1.,0.,0.));
#35653=DIRECTION('ref_axis',(0.,0.,-1.));
#35654=DIRECTION('',(0.,-1.,0.));
#35655=DIRECTION('',(0.,-1.,0.));
#35656=DIRECTION('',(0.,-1.,0.));
#35657=DIRECTION('',(0.,0.,-1.));
#35658=DIRECTION('center_axis',(0.,1.,0.));
#35659=DIRECTION('ref_axis',(0.,0.,1.));
#35660=DIRECTION('',(1.,0.,0.));
#35661=DIRECTION('',(1.,0.,0.));
#35662=DIRECTION('center_axis',(0.,0.,1.));
#35663=DIRECTION('ref_axis',(1.,0.,0.));
#35664=DIRECTION('center_axis',(0.,0.,1.));
#35665=DIRECTION('ref_axis',(1.,0.,0.));
#35666=DIRECTION('center_axis',(0.,0.,1.));
#35667=DIRECTION('ref_axis',(1.,0.,0.));
#35668=DIRECTION('',(1.,0.,0.));
#35669=DIRECTION('center_axis',(0.,1.,0.));
#35670=DIRECTION('ref_axis',(0.,0.,1.));
#35671=DIRECTION('',(1.,0.,0.));
#35672=DIRECTION('',(-1.,0.,0.));
#35673=DIRECTION('center_axis',(0.,0.,-1.));
#35674=DIRECTION('ref_axis',(-1.,0.,0.));
#35675=DIRECTION('',(-1.,0.,0.));
#35676=DIRECTION('center_axis',(-1.,0.,0.));
#35677=DIRECTION('ref_axis',(0.,0.,1.));
#35678=DIRECTION('center_axis',(-1.,0.,0.));
#35679=DIRECTION('ref_axis',(0.,0.,1.));
#66011=CARTESIAN_POINT('',(0.,0.,0.));
#66012=CARTESIAN_POINT('Origin',(-480.,-24.5,0.));
#66013=CARTESIAN_POINT('',(-480.,-7.49999999999999,2.5));
#66014=CARTESIAN_POINT('Origin',(-480.,-7.49999999999999,0.));
#66015=CARTESIAN_POINT('',(-480.,-24.5,2.5));
#66016=CARTESIAN_POINT('',(-480.,-24.5,2.5));
#66017=CARTESIAN_POINT('Origin',(-480.,-24.5,0.));
#66018=CARTESIAN_POINT('Origin',(-480.,-7.49999999999999,0.));
#66019=CARTESIAN_POINT('',(-480.,-5.99784845243109,0.));
#66020=CARTESIAN_POINT('',(-480.,-7.49999999999999,2.5));
#66021=CARTESIAN_POINT('Origin',(-420.,-24.5,0.));
#66022=CARTESIAN_POINT('',(-420.,-7.49999999999999,2.5));
#66023=CARTESIAN_POINT('Origin',(-420.,-7.49999999999999,0.));
#66024=CARTESIAN_POINT('',(-420.,-24.5,2.5));
#66025=CARTESIAN_POINT('',(-420.,-24.5,2.5));
#66026=CARTESIAN_POINT('Origin',(-420.,-24.5,0.));
#66027=CARTESIAN_POINT('Origin',(-420.,-7.49999999999999,0.));
#66028=CARTESIAN_POINT('',(-420.,-5.99784845243109,0.));
#66029=CARTESIAN_POINT('',(-420.,-7.49999999999999,2.5));
#66030=CARTESIAN_POINT('Origin',(-360.,-24.5,0.));
#66031=CARTESIAN_POINT('',(-360.,-7.49999999999999,2.5));
#66032=CARTESIAN_POINT('Origin',(-360.,-7.49999999999999,0.));
#66033=CARTESIAN_POINT('',(-360.,-24.5,2.5));
#66034=CARTESIAN_POINT('',(-360.,-24.5,2.5));
#66035=CARTESIAN_POINT('Origin',(-360.,-24.5,0.));
#66036=CARTESIAN_POINT('Origin',(-360.,-7.49999999999999,0.));
#66037=CARTESIAN_POINT('',(-360.,-5.99784845243109,0.));
#66038=CARTESIAN_POINT('',(-360.,-7.49999999999999,2.5));
#66039=CARTESIAN_POINT('Origin',(-300.,-24.5,0.));
#66040=CARTESIAN_POINT('',(-300.,-7.49999999999999,2.5));
#66041=CARTESIAN_POINT('Origin',(-300.,-7.49999999999999,0.));
#66042=CARTESIAN_POINT('',(-300.,-24.5,2.5));
#66043=CARTESIAN_POINT('',(-300.,-24.5,2.5));
#66044=CARTESIAN_POINT('Origin',(-300.,-24.5,0.));
#66045=CARTESIAN_POINT('Origin',(-300.,-7.49999999999999,0.));
#66046=CARTESIAN_POINT('',(-300.,-5.99784845243109,0.));
#66047=CARTESIAN_POINT('',(-300.,-7.49999999999999,2.5));
#66048=CARTESIAN_POINT('Origin',(-240.,-24.5,0.));
#66049=CARTESIAN_POINT('',(-240.,-7.49999999999999,2.5));
#66050=CARTESIAN_POINT('Origin',(-240.,-7.49999999999999,0.));
#66051=CARTESIAN_POINT('',(-240.,-24.5,2.5));
#66052=CARTESIAN_POINT('',(-240.,-24.5,2.5));
#66053=CARTESIAN_POINT('Origin',(-240.,-24.5,0.));
#66054=CARTESIAN_POINT('Origin',(-240.,-7.49999999999999,0.));
#66055=CARTESIAN_POINT('',(-240.,-5.99784845243109,0.));
#66056=CARTESIAN_POINT('',(-240.,-7.49999999999999,2.5));
#66057=CARTESIAN_POINT('Origin',(-180.,-24.5,0.));
#66058=CARTESIAN_POINT('',(-180.,-7.49999999999999,2.5));
#66059=CARTESIAN_POINT('Origin',(-180.,-7.49999999999999,0.));
#66060=CARTESIAN_POINT('',(-180.,-24.5,2.5));
#66061=CARTESIAN_POINT('',(-180.,-24.5,2.5));
#66062=CARTESIAN_POINT('Origin',(-180.,-24.5,0.));
#66063=CARTESIAN_POINT('Origin',(-180.,-7.49999999999999,0.));
#66064=CARTESIAN_POINT('',(-180.,-5.99784845243109,0.));
#66065=CARTESIAN_POINT('',(-180.,-7.49999999999999,2.5));
#66066=CARTESIAN_POINT('Origin',(-120.,-24.5,0.));
#66067=CARTESIAN_POINT('',(-120.,-7.49999999999999,2.5));
#66068=CARTESIAN_POINT('Origin',(-120.,-7.49999999999999,0.));
#66069=CARTESIAN_POINT('',(-120.,-24.5,2.5));
#66070=CARTESIAN_POINT('',(-120.,-24.5,2.5));
#66071=CARTESIAN_POINT('Origin',(-120.,-24.5,0.));
#66072=CARTESIAN_POINT('Origin',(-120.,-7.49999999999999,0.));
#66073=CARTESIAN_POINT('',(-120.,-5.99784845243109,0.));
#66074=CARTESIAN_POINT('',(-120.,-7.49999999999999,2.5));
#66075=CARTESIAN_POINT('Origin',(-60.,-24.5,0.));
#66076=CARTESIAN_POINT('',(-60.,-7.49999999999999,2.5));
#66077=CARTESIAN_POINT('Origin',(-60.,-7.49999999999999,0.));
#66078=CARTESIAN_POINT('',(-60.,-24.5,2.5));
#66079=CARTESIAN_POINT('',(-60.,-24.5,2.5));
#66080=CARTESIAN_POINT('Origin',(-60.,-24.5,0.));
#66081=CARTESIAN_POINT('Origin',(-60.,-7.49999999999999,0.));
#66082=CARTESIAN_POINT('',(-60.,-5.99784845243109,0.));
#66083=CARTESIAN_POINT('',(-60.,-7.49999999999999,2.5));
#66084=CARTESIAN_POINT('Origin',(480.,-24.5,0.));
#66085=CARTESIAN_POINT('',(480.,-7.49999999999999,2.5));
#66086=CARTESIAN_POINT('Origin',(480.,-7.49999999999999,0.));
#66087=CARTESIAN_POINT('',(480.,-24.5,2.5));
#66088=CARTESIAN_POINT('',(480.,-24.5,2.5));
#66089=CARTESIAN_POINT('Origin',(480.,-24.5,0.));
#66090=CARTESIAN_POINT('Origin',(480.,-7.49999999999999,0.));
#66091=CARTESIAN_POINT('',(480.,-5.99784845243109,0.));
#66092=CARTESIAN_POINT('',(480.,-7.49999999999999,2.5));
#66093=CARTESIAN_POINT('Origin',(420.,-24.5,0.));
#66094=CARTESIAN_POINT('',(420.,-7.49999999999999,2.5));
#66095=CARTESIAN_POINT('Origin',(420.,-7.49999999999999,0.));
#66096=CARTESIAN_POINT('',(420.,-24.5,2.5));
#66097=CARTESIAN_POINT('',(420.,-24.5,2.5));
#66098=CARTESIAN_POINT('Origin',(420.,-24.5,0.));
#66099=CARTESIAN_POINT('Origin',(420.,-7.49999999999999,0.));
#66100=CARTESIAN_POINT('',(420.,-5.99784845243109,0.));
#66101=CARTESIAN_POINT('',(420.,-7.49999999999999,2.5));
#66102=CARTESIAN_POINT('Origin',(360.,-24.5,0.));
#66103=CARTESIAN_POINT('',(360.,-7.49999999999999,2.5));
#66104=CARTESIAN_POINT('Origin',(360.,-7.49999999999999,0.));
#66105=CARTESIAN_POINT('',(360.,-24.5,2.5));
#66106=CARTESIAN_POINT('',(360.,-24.5,2.5));
#66107=CARTESIAN_POINT('Origin',(360.,-24.5,0.));
#66108=CARTESIAN_POINT('Origin',(360.,-7.49999999999999,0.));
#66109=CARTESIAN_POINT('',(360.,-5.99784845243109,0.));
#66110=CARTESIAN_POINT('',(360.,-7.49999999999999,2.5));
#66111=CARTESIAN_POINT('Origin',(300.,-24.5,0.));
#66112=CARTESIAN_POINT('',(300.,-7.49999999999999,2.5));
#66113=CARTESIAN_POINT('Origin',(300.,-7.49999999999999,0.));
#66114=CARTESIAN_POINT('',(300.,-24.5,2.5));
#66115=CARTESIAN_POINT('',(300.,-24.5,2.5));
#66116=CARTESIAN_POINT('Origin',(300.,-24.5,0.));
#66117=CARTESIAN_POINT('Origin',(300.,-7.49999999999999,0.));
#66118=CARTESIAN_POINT('',(300.,-5.99784845243109,0.));
#66119=CARTESIAN_POINT('',(300.,-7.49999999999999,2.5));
#66120=CARTESIAN_POINT('Origin',(240.,-24.5,0.));
#66121=CARTESIAN_POINT('',(240.,-7.49999999999999,2.5));
#66122=CARTESIAN_POINT('Origin',(240.,-7.49999999999999,0.));
#66123=CARTESIAN_POINT('',(240.,-24.5,2.5));
#66124=CARTESIAN_POINT('',(240.,-24.5,2.5));
#66125=CARTESIAN_POINT('Origin',(240.,-24.5,0.));
#66126=CARTESIAN_POINT('Origin',(240.,-7.49999999999999,0.));
#66127=CARTESIAN_POINT('',(240.,-5.99784845243109,0.));
#66128=CARTESIAN_POINT('',(240.,-7.49999999999999,2.5));
#66129=CARTESIAN_POINT('Origin',(180.,-24.5,0.));
#66130=CARTESIAN_POINT('',(180.,-7.49999999999999,2.5));
#66131=CARTESIAN_POINT('Origin',(180.,-7.49999999999999,0.));
#66132=CARTESIAN_POINT('',(180.,-24.5,2.5));
#66133=CARTESIAN_POINT('',(180.,-24.5,2.5));
#66134=CARTESIAN_POINT('Origin',(180.,-24.5,0.));
#66135=CARTESIAN_POINT('Origin',(180.,-7.49999999999999,0.));
#66136=CARTESIAN_POINT('',(180.,-5.99784845243109,0.));
#66137=CARTESIAN_POINT('',(180.,-7.49999999999999,2.5));
#66138=CARTESIAN_POINT('Origin',(120.,-24.5,0.));
#66139=CARTESIAN_POINT('',(120.,-7.49999999999999,2.5));
#66140=CARTESIAN_POINT('Origin',(120.,-7.49999999999999,0.));
#66141=CARTESIAN_POINT('',(120.,-24.5,2.5));
#66142=CARTESIAN_POINT('',(120.,-24.5,2.5));
#66143=CARTESIAN_POINT('Origin',(120.,-24.5,0.));
#66144=CARTESIAN_POINT('Origin',(120.,-7.49999999999999,0.));
#66145=CARTESIAN_POINT('',(120.,-5.99784845243109,0.));
#66146=CARTESIAN_POINT('',(120.,-7.49999999999999,2.5));
#66147=CARTESIAN_POINT('Origin',(60.,-24.5,0.));
#66148=CARTESIAN_POINT('',(60.,-7.49999999999999,2.5));
#66149=CARTESIAN_POINT('Origin',(60.,-7.49999999999999,0.));
#66150=CARTESIAN_POINT('',(60.,-24.5,2.5));
#66151=CARTESIAN_POINT('',(60.,-24.5,2.5));
#66152=CARTESIAN_POINT('Origin',(60.,-24.5,0.));
#66153=CARTESIAN_POINT('Origin',(60.,-7.49999999999999,0.));
#66154=CARTESIAN_POINT('',(60.,-5.99784845243109,0.));
#66155=CARTESIAN_POINT('',(60.,-7.49999999999999,2.5));
#66156=CARTESIAN_POINT('Origin',(0.,-24.5,0.));
#66157=CARTESIAN_POINT('',(-3.06161699786838E-16,-7.49999999999999,2.5));
#66158=CARTESIAN_POINT('Origin',(0.,-7.49999999999999,0.));
#66159=CARTESIAN_POINT('',(-3.06161699786838E-16,-24.5,2.5));
#66160=CARTESIAN_POINT('',(-3.06161699786838E-16,-24.5,2.5));
#66161=CARTESIAN_POINT('Origin',(0.,-24.5,0.));
#66162=CARTESIAN_POINT('Origin',(0.,-7.49999999999999,0.));
#66163=CARTESIAN_POINT('',(-4.5317201340139E-15,-5.99784845243109,0.));
#66164=CARTESIAN_POINT('',(-3.06161699786838E-16,-7.49999999999999,2.5));
#66165=CARTESIAN_POINT('Origin',(-515.,-26.5,17.5));
#66166=CARTESIAN_POINT('',(-515.,-26.5,17.5));
#66167=CARTESIAN_POINT('',(-515.,-26.5,11.5));
#66168=CARTESIAN_POINT('',(-515.,-26.5,17.5));
#66169=CARTESIAN_POINT('',(515.,-26.5,11.5));
#66170=CARTESIAN_POINT('',(-515.,-26.5,11.5));
#66171=CARTESIAN_POINT('',(515.,-26.5,17.5));
#66172=CARTESIAN_POINT('',(515.,-26.5,17.5));
#66173=CARTESIAN_POINT('',(-515.,-26.5,17.5));
#66174=CARTESIAN_POINT('Origin',(515.,26.5,17.5));
#66175=CARTESIAN_POINT('',(515.,-24.7,11.5));
#66176=CARTESIAN_POINT('',(515.,-26.5,11.5));
#66177=CARTESIAN_POINT('',(515.,-24.5,11.3));
#66178=CARTESIAN_POINT('Origin',(515.,-24.7,11.3));
#66179=CARTESIAN_POINT('',(515.,-24.5,-11.3));
#66180=CARTESIAN_POINT('',(515.,-24.5,11.5));
#66181=CARTESIAN_POINT('',(515.,-24.7,-11.5));
#66182=CARTESIAN_POINT('Origin',(515.,-24.7,-11.3));
#66183=CARTESIAN_POINT('',(515.,-26.5,-11.5));
#66184=CARTESIAN_POINT('',(515.,-26.5,-11.5));
#66185=CARTESIAN_POINT('',(515.,-26.5,-17.5));
#66186=CARTESIAN_POINT('',(515.,-26.5,17.5));
#66187=CARTESIAN_POINT('',(515.,26.5,-17.5));
#66188=CARTESIAN_POINT('',(515.,26.5,-17.5));
#66189=CARTESIAN_POINT('',(515.,26.5,17.5));
#66190=CARTESIAN_POINT('',(515.,26.5,17.5));
#66191=CARTESIAN_POINT('',(515.,26.5,17.5));
#66192=CARTESIAN_POINT('Origin',(-515.,26.5,17.5));
#66193=CARTESIAN_POINT('',(-515.,26.5,-17.5));
#66194=CARTESIAN_POINT('',(-515.,26.5,-17.5));
#66195=CARTESIAN_POINT('',(-515.,26.5,17.5));
#66196=CARTESIAN_POINT('',(-515.,26.5,17.5));
#66197=CARTESIAN_POINT('',(-515.,26.5,17.5));
#66198=CARTESIAN_POINT('Origin',(-515.,26.5,17.5));
#66199=CARTESIAN_POINT('',(-515.,-26.5,-11.5));
#66200=CARTESIAN_POINT('',(-515.,-24.7,-11.5));
#66201=CARTESIAN_POINT('',(-515.,-26.5,-11.5));
#66202=CARTESIAN_POINT('',(-515.,-24.5,-11.3));
#66203=CARTESIAN_POINT('Origin',(-515.,-24.7,-11.3));
#66204=CARTESIAN_POINT('',(-515.,-24.5,11.3));
#66205=CARTESIAN_POINT('',(-515.,-24.5,11.5));
#66206=CARTESIAN_POINT('',(-515.,-24.7,11.5));
#66207=CARTESIAN_POINT('Origin',(-515.,-24.7,11.3));
#66208=CARTESIAN_POINT('',(-515.,-26.5,11.5));
#66209=CARTESIAN_POINT('',(-515.,26.5,17.5));
#66210=CARTESIAN_POINT('',(-515.,-26.5,-17.5));
#66211=CARTESIAN_POINT('',(-515.,26.5,-17.5));
#66212=CARTESIAN_POINT('',(-515.,-26.5,17.5));
#66213=CARTESIAN_POINT('Origin',(-515.,-26.5,17.5));
#66214=CARTESIAN_POINT('',(-515.,-26.5,-11.5));
#66215=CARTESIAN_POINT('',(-515.,-26.5,-17.5));
#66216=CARTESIAN_POINT('Origin',(0.,0.,17.5));
#66217=CARTESIAN_POINT('Origin',(0.,0.,-17.5));
#66218=CARTESIAN_POINT('Origin',(-515.,-26.5,11.5));
#66219=CARTESIAN_POINT('',(515.,-24.7,11.5));
#66220=CARTESIAN_POINT('Origin',(-515.,-24.5,11.5));
#66221=CARTESIAN_POINT('',(515.,-24.5,-11.3));
#66222=CARTESIAN_POINT('',(-515.,-24.5,11.3));
#66223=CARTESIAN_POINT('Origin',(-515.,-26.5,-11.5));
#66224=CARTESIAN_POINT('',(-515.,-24.7,-11.5));
#66225=CARTESIAN_POINT('Origin',(-515.,-24.7,-11.3));
#66226=CARTESIAN_POINT('Origin',(-515.,-24.7,11.3));
#66675=UNCERTAINTY_MEASURE_WITH_UNIT(LENGTH_MEASURE(0.01),#66722,
'DISTANCE_ACCURACY_VALUE',
'Maximum model space distance between geometric entities at asserted c
onnectivities');
#66680=UNCERTAINTY_MEASURE_WITH_UNIT(LENGTH_MEASURE(0.01),#66722,
'DISTANCE_ACCURACY_VALUE',
'Maximum model space distance between geometric entities at asserted c
onnectivities');
#66716=(
GEOMETRIC_REPRESENTATION_CONTEXT(3)
GLOBAL_UNCERTAINTY_ASSIGNED_CONTEXT((#66675))
GLOBAL_UNIT_ASSIGNED_CONTEXT((#66722,#66724,#66725))
REPRESENTATION_CONTEXT('','3D')
);
#66721=(
GEOMETRIC_REPRESENTATION_CONTEXT(3)
GLOBAL_UNCERTAINTY_ASSIGNED_CONTEXT((#66680))
GLOBAL_UNIT_ASSIGNED_CONTEXT((#66722,#66724,#66725))
REPRESENTATION_CONTEXT('','3D')
);
#66722=(
LENGTH_UNIT()
NAMED_UNIT(*)
SI_UNIT(.MILLI.,.METRE.)
);
#66724=(
NAMED_UNIT(*)
PLANE_ANGLE_UNIT()
SI_UNIT($,.RADIAN.)
);
#66725=(
NAMED_UNIT(*)
SI_UNIT($,.STERADIAN.)
SOLID_ANGLE_UNIT()
);
#66761=SHAPE_DEFINITION_REPRESENTATION(#66831,#66925);
#66831=PRODUCT_DEFINITION_SHAPE('',$,#66966);
#66925=SHAPE_REPRESENTATION('',(#28479),#66716);
#66930=PRODUCT_DEFINITION_CONTEXT('part definition',#67052,'design');
#66966=PRODUCT_DEFINITION('Linear Guide Spacer','Linear Guide Spacer',#67006,
#66930);
#67006=PRODUCT_DEFINITION_FORMATION('',$,#67089);
#67052=APPLICATION_CONTEXT(
'Core Data for Automotive Mechanical Design Process');
#67053=PRODUCT_CONTEXT('part definition',#67052,'mechanical');
#67089=PRODUCT('Linear Guide Spacer','Linear Guide Spacer',$,(#67053));
#67095=PRESENTATION_STYLE_ASSIGNMENT((#67097));
#67097=SURFACE_STYLE_USAGE(.BOTH.,#67099);
#67099=SURFACE_SIDE_STYLE('',(#67101));
#67101=SURFACE_STYLE_FILL_AREA(#67103);
#67103=FILL_AREA_STYLE('Opaque(202,209,238)',(#67105));
#67105=FILL_AREA_STYLE_COLOUR('Opaque(202,209,238)',#67107);
#67107=COLOUR_RGB('Opaque(202,209,238)',0.792156862745098,0.819607843137255,
0.933333333333333);
ENDSEC;
END-ISO-10303-21;
